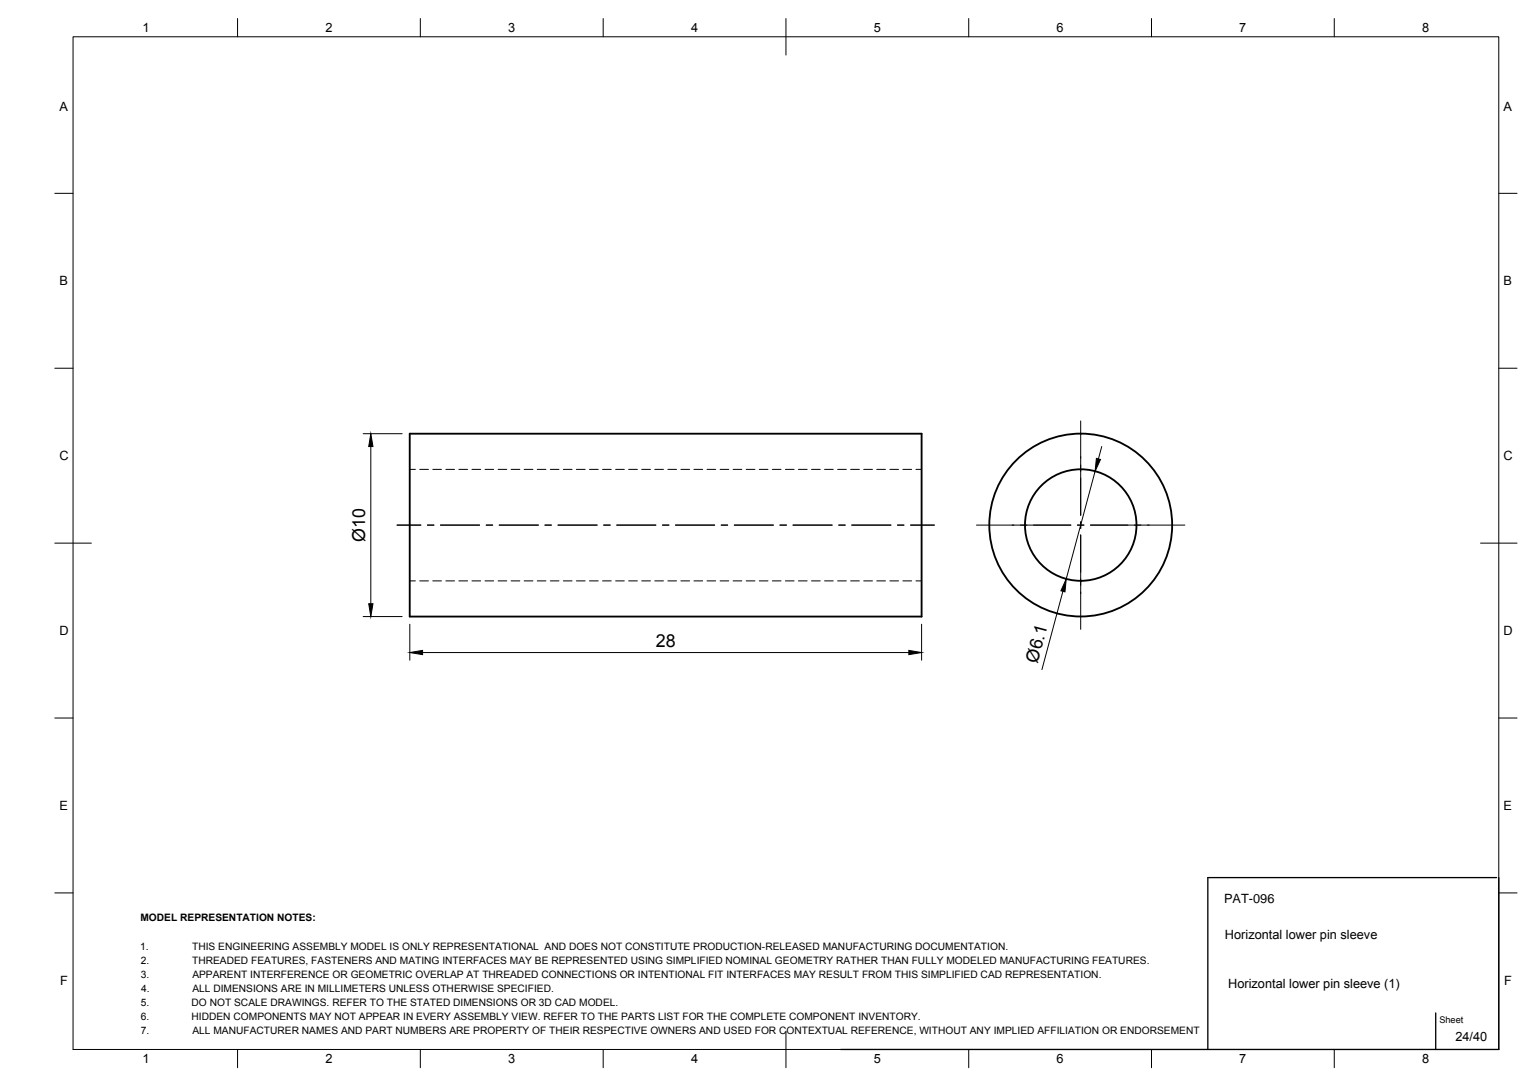
ISO-10303-21;
HEADER;
/* Generated by software containing ST-Developer
 * from STEP Tools, Inc. (www.steptools.com) 
 */

FILE_DESCRIPTION(
/* description */ ('PAT-096'),
/* implementation_level */ '2;1');

FILE_NAME(
/* name */ 'Horizontal lower pin sleeve.step',
/* time_stamp */ '2026-10-29T17:03:14-07:00',
/* author */ (''),
/* organization */ (''),
/* preprocessor_version */ 'ST-DEVELOPER v20.2',
/* originating_system */ 'Autodesk Translation Framework v15.17.0.0',
/* authorisation */ '');

FILE_SCHEMA (('AUTOMOTIVE_DESIGN { 1 0 10303 214 3 1 1 }'));
ENDSEC;

DATA;
#10=MECHANICAL_DESIGN_GEOMETRIC_PRESENTATION_REPRESENTATION('',(#425),#10650);
#355=SHAPE_REPRESENTATION_RELATIONSHIP('SRR','None',#10817,#386);
#386=ADVANCED_BREP_SHAPE_REPRESENTATION('',(#462),#10635);
#425=STYLED_ITEM('',(#11064),#462);
#462=MANIFOLD_SOLID_BREP('Body1',#5560);
#562=FACE_BOUND('',#1452,.T.);
#563=FACE_BOUND('',#1454,.T.);
#730=PLANE('',#6416);
#731=PLANE('',#6417);
#1024=FACE_OUTER_BOUND('',#1449,.T.);
#1025=FACE_OUTER_BOUND('',#1450,.T.);
#1026=FACE_OUTER_BOUND('',#1451,.T.);
#1027=FACE_OUTER_BOUND('',#1453,.T.);
#1449=EDGE_LOOP('',(#4683,#4684,#4685,#4686));
#1450=EDGE_LOOP('',(#4687,#4688,#4689,#4690));
#1451=EDGE_LOOP('',(#4691));
#1452=EDGE_LOOP('',(#4692));
#1453=EDGE_LOOP('',(#4693));
#1454=EDGE_LOOP('',(#4694));
#1822=LINE('',#10079,#2151);
#1823=LINE('',#10085,#2152);
#2151=VECTOR('',#7886,0.305);
#2152=VECTOR('',#7893,0.5);
#2491=CIRCLE('',#6411,0.305);
#2492=CIRCLE('',#6412,0.305);
#2493=CIRCLE('',#6414,0.5);
#2494=CIRCLE('',#6415,0.5);
#2907=VERTEX_POINT('',#10076);
#2908=VERTEX_POINT('',#10078);
#2909=VERTEX_POINT('',#10082);
#2910=VERTEX_POINT('',#10084);
#3520=EDGE_CURVE('',#2907,#2907,#2491,.T.);
#3521=EDGE_CURVE('',#2907,#2908,#1822,.T.);
#3522=EDGE_CURVE('',#2908,#2908,#2492,.T.);
#3523=EDGE_CURVE('',#2909,#2909,#2493,.T.);
#3524=EDGE_CURVE('',#2909,#2910,#1823,.T.);
#3525=EDGE_CURVE('',#2910,#2910,#2494,.T.);
#4683=ORIENTED_EDGE('',*,*,#3520,.F.);
#4684=ORIENTED_EDGE('',*,*,#3521,.T.);
#4685=ORIENTED_EDGE('',*,*,#3522,.T.);
#4686=ORIENTED_EDGE('',*,*,#3521,.F.);
#4687=ORIENTED_EDGE('',*,*,#3523,.F.);
#4688=ORIENTED_EDGE('',*,*,#3524,.T.);
#4689=ORIENTED_EDGE('',*,*,#3525,.T.);
#4690=ORIENTED_EDGE('',*,*,#3524,.F.);
#4691=ORIENTED_EDGE('',*,*,#3523,.T.);
#4692=ORIENTED_EDGE('',*,*,#3520,.T.);
#4693=ORIENTED_EDGE('',*,*,#3525,.F.);
#4694=ORIENTED_EDGE('',*,*,#3522,.F.);
#5156=CYLINDRICAL_SURFACE('',#6410,0.305);
#5157=CYLINDRICAL_SURFACE('',#6413,0.5);
#5429=ADVANCED_FACE('',(#1024),#5156,.F.);
#5430=ADVANCED_FACE('',(#1025),#5157,.T.);
#5431=ADVANCED_FACE('',(#1026,#562),#730,.T.);
#5432=ADVANCED_FACE('',(#1027,#563),#731,.F.);
#5560=CLOSED_SHELL('',(#5429,#5430,#5431,#5432));
#6409=AXIS2_PLACEMENT_3D('',#10074,#7880,#7881);
#6410=AXIS2_PLACEMENT_3D('',#10075,#7882,#7883);
#6411=AXIS2_PLACEMENT_3D('',#10077,#7884,#7885);
#6412=AXIS2_PLACEMENT_3D('',#10080,#7887,#7888);
#6413=AXIS2_PLACEMENT_3D('',#10081,#7889,#7890);
#6414=AXIS2_PLACEMENT_3D('',#10083,#7891,#7892);
#6415=AXIS2_PLACEMENT_3D('',#10086,#7894,#7895);
#6416=AXIS2_PLACEMENT_3D('',#10087,#7896,#7897);
#6417=AXIS2_PLACEMENT_3D('',#10088,#7898,#7899);
#7880=DIRECTION('axis',(0.,0.,1.));
#7881=DIRECTION('refdir',(1.,0.,0.));
#7882=DIRECTION('center_axis',(0.,0.,1.));
#7883=DIRECTION('ref_axis',(1.,0.,0.));
#7884=DIRECTION('center_axis',(0.,0.,-1.));
#7885=DIRECTION('ref_axis',(1.,0.,0.));
#7886=DIRECTION('',(0.,0.,-1.));
#7887=DIRECTION('center_axis',(0.,0.,-1.));
#7888=DIRECTION('ref_axis',(1.,0.,0.));
#7889=DIRECTION('center_axis',(0.,0.,1.));
#7890=DIRECTION('ref_axis',(1.,0.,0.));
#7891=DIRECTION('center_axis',(0.,0.,1.));
#7892=DIRECTION('ref_axis',(1.,0.,0.));
#7893=DIRECTION('',(0.,0.,-1.));
#7894=DIRECTION('center_axis',(0.,0.,1.));
#7895=DIRECTION('ref_axis',(1.,0.,0.));
#7896=DIRECTION('center_axis',(0.,0.,1.));
#7897=DIRECTION('ref_axis',(1.,0.,0.));
#7898=DIRECTION('center_axis',(0.,0.,1.));
#7899=DIRECTION('ref_axis',(1.,0.,0.));
#10074=CARTESIAN_POINT('',(0.,0.,0.));
#10075=CARTESIAN_POINT('Origin',(0.,2.,6.));
#10076=CARTESIAN_POINT('',(-0.305,2.,8.8));
#10077=CARTESIAN_POINT('Origin',(0.,2.,8.8));
#10078=CARTESIAN_POINT('',(-0.305,2.,6.));
#10079=CARTESIAN_POINT('',(-0.305,2.,6.));
#10080=CARTESIAN_POINT('Origin',(0.,2.,6.));
#10081=CARTESIAN_POINT('Origin',(0.,2.,6.));
#10082=CARTESIAN_POINT('',(-0.5,2.,8.8));
#10083=CARTESIAN_POINT('Origin',(0.,2.,8.8));
#10084=CARTESIAN_POINT('',(-0.5,2.,6.));
#10085=CARTESIAN_POINT('',(-0.5,2.,6.));
#10086=CARTESIAN_POINT('Origin',(0.,2.,6.));
#10087=CARTESIAN_POINT('Origin',(0.,2.,8.8));
#10088=CARTESIAN_POINT('Origin',(0.,2.,6.));
#10596=UNCERTAINTY_MEASURE_WITH_UNIT(LENGTH_MEASURE(0.001),#10651,
'DISTANCE_ACCURACY_VALUE',
'Maximum model space distance between geometric entities at asserted c
onnectivities');
#10611=UNCERTAINTY_MEASURE_WITH_UNIT(LENGTH_MEASURE(0.001),#10651,
'DISTANCE_ACCURACY_VALUE',
'Maximum model space distance between geometric entities at asserted c
onnectivities');
#10635=(
GEOMETRIC_REPRESENTATION_CONTEXT(3)
GLOBAL_UNCERTAINTY_ASSIGNED_CONTEXT((#10596))
GLOBAL_UNIT_ASSIGNED_CONTEXT((#10651,#10653,#10654))
REPRESENTATION_CONTEXT('','3D')
);
#10650=(
GEOMETRIC_REPRESENTATION_CONTEXT(3)
GLOBAL_UNCERTAINTY_ASSIGNED_CONTEXT((#10611))
GLOBAL_UNIT_ASSIGNED_CONTEXT((#10651,#10653,#10654))
REPRESENTATION_CONTEXT('','3D')
);
#10651=(
LENGTH_UNIT()
NAMED_UNIT(*)
SI_UNIT(.CENTI.,.METRE.)
);
#10653=(
NAMED_UNIT(*)
PLANE_ANGLE_UNIT()
SI_UNIT($,.RADIAN.)
);
#10654=(
NAMED_UNIT(*)
SI_UNIT($,.STERADIAN.)
SOLID_ANGLE_UNIT()
);
#10678=SHAPE_DEFINITION_REPRESENTATION(#10721,#10817);
#10721=PRODUCT_DEFINITION_SHAPE('',$,#10856);
#10817=SHAPE_REPRESENTATION('',(#6409),#10635);
#10832=PRODUCT_DEFINITION_CONTEXT('part definition',#10948,'design');
#10856=PRODUCT_DEFINITION('Horizontal lower pin sleeve',
'Horizontal lower pin sleeve',#10894,#10832);
#10894=PRODUCT_DEFINITION_FORMATION('',$,#10973);
#10948=APPLICATION_CONTEXT(
'Core Data for Automotive Mechanical Design Process');
#10949=PRODUCT_CONTEXT('part definition',#10948,'mechanical');
#10973=PRODUCT('Horizontal lower pin sleeve',
'Horizontal lower pin sleeve','Horizontal lower pin sleeve',(#10949));
#11058=COLOUR_RGB('Grey',0.48,0.52,0.57);
#11059=FILL_AREA_STYLE_COLOUR('',#11058);
#11060=FILL_AREA_STYLE('',(#11059));
#11061=SURFACE_STYLE_FILL_AREA(#11060);
#11062=SURFACE_SIDE_STYLE('',(#11061));
#11063=SURFACE_STYLE_USAGE(.BOTH.,#11062);
#11064=PRESENTATION_STYLE_ASSIGNMENT((#11063));
ENDSEC;
END-ISO-10303-21;
